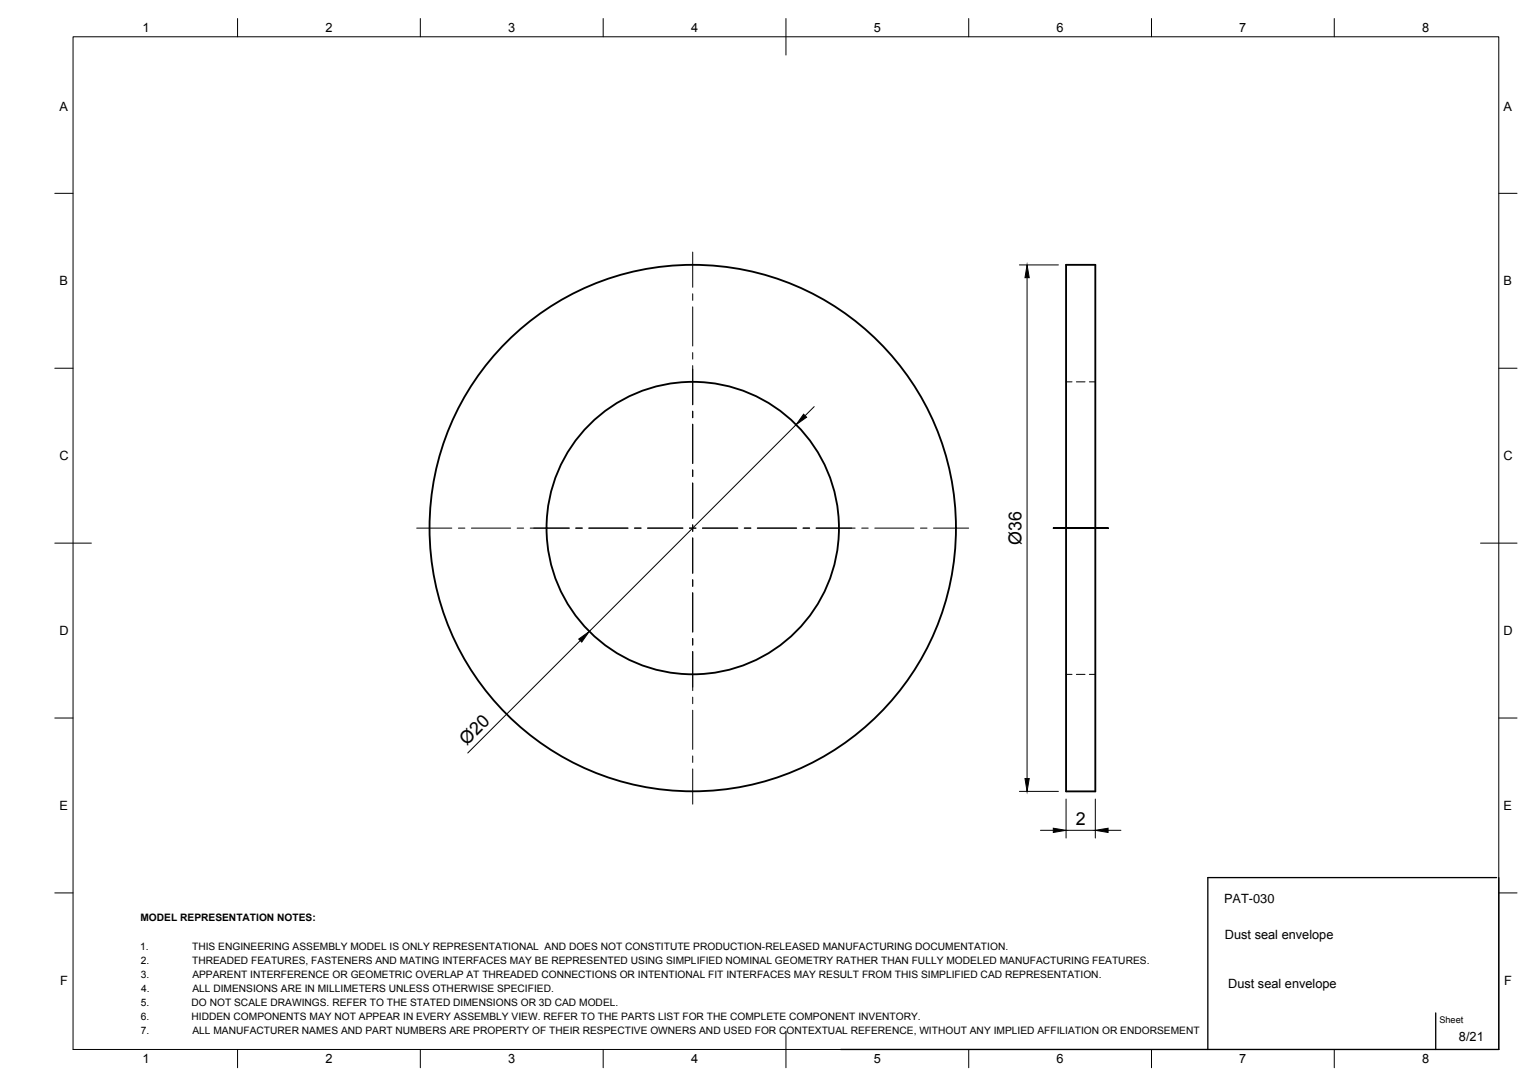
ISO-10303-21;
HEADER;
/* Generated by software containing ST-Developer
 * from STEP Tools, Inc. (www.steptools.com) 
 */

FILE_DESCRIPTION(
/* description */ ('Double-bearing flanged cartridge'),
/* implementation_level */ '2;1');

FILE_NAME(
/* name */ 'Dust seal envelope.step',
/* time_stamp */ '2026-10-28T03:26:40-07:00',
/* author */ (''),
/* organization */ (''),
/* preprocessor_version */ 'ST-DEVELOPER v20.2',
/* originating_system */ 'Autodesk Translation Framework v15.17.0.0',
/* authorisation */ '');

FILE_SCHEMA (('AUTOMOTIVE_DESIGN { 1 0 10303 214 3 1 1 }'));
ENDSEC;

DATA;
#10=MECHANICAL_DESIGN_GEOMETRIC_PRESENTATION_REPRESENTATION('',(#206),#5535);
#170=SHAPE_REPRESENTATION_RELATIONSHIP('SRR','None',#5612,#184);
#184=ADVANCED_BREP_SHAPE_REPRESENTATION('',(#228),#5528);
#206=STYLED_ITEM('',(#5771),#228);
#228=MANIFOLD_SOLID_BREP('Body1',#2340);
#276=FACE_BOUND('',#651,.T.);
#277=FACE_BOUND('',#653,.T.);
#335=PLANE('',#2744);
#336=PLANE('',#2745);
#456=FACE_OUTER_BOUND('',#648,.T.);
#457=FACE_OUTER_BOUND('',#649,.T.);
#458=FACE_OUTER_BOUND('',#650,.T.);
#459=FACE_OUTER_BOUND('',#652,.T.);
#648=EDGE_LOOP('',(#1918,#1919,#1920,#1921));
#649=EDGE_LOOP('',(#1922,#1923,#1924,#1925));
#650=EDGE_LOOP('',(#1926));
#651=EDGE_LOOP('',(#1927));
#652=EDGE_LOOP('',(#1928));
#653=EDGE_LOOP('',(#1929));
#768=LINE('',#4453,#854);
#769=LINE('',#4459,#855);
#854=VECTOR('',#3385,1.);
#855=VECTOR('',#3392,1.8);
#1022=CIRCLE('',#2739,1.);
#1023=CIRCLE('',#2740,1.);
#1024=CIRCLE('',#2742,1.8);
#1025=CIRCLE('',#2743,1.8);
#1204=VERTEX_POINT('',#4450);
#1205=VERTEX_POINT('',#4452);
#1206=VERTEX_POINT('',#4456);
#1207=VERTEX_POINT('',#4458);
#1452=EDGE_CURVE('',#1204,#1204,#1022,.T.);
#1453=EDGE_CURVE('',#1204,#1205,#768,.T.);
#1454=EDGE_CURVE('',#1205,#1205,#1023,.T.);
#1455=EDGE_CURVE('',#1206,#1206,#1024,.T.);
#1456=EDGE_CURVE('',#1206,#1207,#769,.T.);
#1457=EDGE_CURVE('',#1207,#1207,#1025,.T.);
#1918=ORIENTED_EDGE('',*,*,#1452,.F.);
#1919=ORIENTED_EDGE('',*,*,#1453,.T.);
#1920=ORIENTED_EDGE('',*,*,#1454,.T.);
#1921=ORIENTED_EDGE('',*,*,#1453,.F.);
#1922=ORIENTED_EDGE('',*,*,#1455,.F.);
#1923=ORIENTED_EDGE('',*,*,#1456,.T.);
#1924=ORIENTED_EDGE('',*,*,#1457,.T.);
#1925=ORIENTED_EDGE('',*,*,#1456,.F.);
#1926=ORIENTED_EDGE('',*,*,#1455,.T.);
#1927=ORIENTED_EDGE('',*,*,#1452,.T.);
#1928=ORIENTED_EDGE('',*,*,#1457,.F.);
#1929=ORIENTED_EDGE('',*,*,#1454,.F.);
#2152=CYLINDRICAL_SURFACE('',#2738,1.);
#2153=CYLINDRICAL_SURFACE('',#2741,1.8);
#2270=ADVANCED_FACE('',(#456),#2152,.F.);
#2271=ADVANCED_FACE('',(#457),#2153,.T.);
#2272=ADVANCED_FACE('',(#458,#276),#335,.T.);
#2273=ADVANCED_FACE('',(#459,#277),#336,.F.);
#2340=CLOSED_SHELL('',(#2270,#2271,#2272,#2273));
#2737=AXIS2_PLACEMENT_3D('',#4448,#3379,#3380);
#2738=AXIS2_PLACEMENT_3D('',#4449,#3381,#3382);
#2739=AXIS2_PLACEMENT_3D('',#4451,#3383,#3384);
#2740=AXIS2_PLACEMENT_3D('',#4454,#3386,#3387);
#2741=AXIS2_PLACEMENT_3D('',#4455,#3388,#3389);
#2742=AXIS2_PLACEMENT_3D('',#4457,#3390,#3391);
#2743=AXIS2_PLACEMENT_3D('',#4460,#3393,#3394);
#2744=AXIS2_PLACEMENT_3D('',#4461,#3395,#3396);
#2745=AXIS2_PLACEMENT_3D('',#4462,#3397,#3398);
#3379=DIRECTION('axis',(0.,0.,1.));
#3380=DIRECTION('refdir',(1.,0.,0.));
#3381=DIRECTION('center_axis',(0.,1.,0.));
#3382=DIRECTION('ref_axis',(1.,0.,0.));
#3383=DIRECTION('center_axis',(0.,-1.,0.));
#3384=DIRECTION('ref_axis',(1.,0.,0.));
#3385=DIRECTION('',(0.,-1.,0.));
#3386=DIRECTION('center_axis',(0.,-1.,0.));
#3387=DIRECTION('ref_axis',(1.,0.,0.));
#3388=DIRECTION('center_axis',(0.,1.,0.));
#3389=DIRECTION('ref_axis',(1.,0.,0.));
#3390=DIRECTION('center_axis',(0.,1.,0.));
#3391=DIRECTION('ref_axis',(1.,0.,0.));
#3392=DIRECTION('',(0.,-1.,0.));
#3393=DIRECTION('center_axis',(0.,1.,0.));
#3394=DIRECTION('ref_axis',(1.,0.,0.));
#3395=DIRECTION('center_axis',(0.,1.,0.));
#3396=DIRECTION('ref_axis',(1.,0.,0.));
#3397=DIRECTION('center_axis',(0.,1.,0.));
#3398=DIRECTION('ref_axis',(1.,0.,0.));
#4448=CARTESIAN_POINT('',(0.,0.,0.));
#4449=CARTESIAN_POINT('Origin',(0.,-0.4,4.5));
#4450=CARTESIAN_POINT('',(-1.,-0.2,4.5));
#4451=CARTESIAN_POINT('Origin',(0.,-0.2,4.5));
#4452=CARTESIAN_POINT('',(-1.,-0.4,4.5));
#4453=CARTESIAN_POINT('',(-1.,-0.4,4.5));
#4454=CARTESIAN_POINT('Origin',(0.,-0.4,4.5));
#4455=CARTESIAN_POINT('Origin',(0.,-0.4,4.5));
#4456=CARTESIAN_POINT('',(-1.8,-0.2,4.5));
#4457=CARTESIAN_POINT('Origin',(0.,-0.2,4.5));
#4458=CARTESIAN_POINT('',(-1.8,-0.4,4.5));
#4459=CARTESIAN_POINT('',(-1.8,-0.4,4.5));
#4460=CARTESIAN_POINT('Origin',(0.,-0.4,4.5));
#4461=CARTESIAN_POINT('Origin',(0.,-0.2,4.5));
#4462=CARTESIAN_POINT('Origin',(0.,-0.4,4.5));
#5509=UNCERTAINTY_MEASURE_WITH_UNIT(LENGTH_MEASURE(0.001),#5536,
'DISTANCE_ACCURACY_VALUE',
'Maximum model space distance between geometric entities at asserted c
onnectivities');
#5516=UNCERTAINTY_MEASURE_WITH_UNIT(LENGTH_MEASURE(0.001),#5536,
'DISTANCE_ACCURACY_VALUE',
'Maximum model space distance between geometric entities at asserted c
onnectivities');
#5528=(
GEOMETRIC_REPRESENTATION_CONTEXT(3)
GLOBAL_UNCERTAINTY_ASSIGNED_CONTEXT((#5509))
GLOBAL_UNIT_ASSIGNED_CONTEXT((#5536,#5538,#5539))
REPRESENTATION_CONTEXT('','3D')
);
#5535=(
GEOMETRIC_REPRESENTATION_CONTEXT(3)
GLOBAL_UNCERTAINTY_ASSIGNED_CONTEXT((#5516))
GLOBAL_UNIT_ASSIGNED_CONTEXT((#5536,#5538,#5539))
REPRESENTATION_CONTEXT('','3D')
);
#5536=(
LENGTH_UNIT()
NAMED_UNIT(*)
SI_UNIT(.CENTI.,.METRE.)
);
#5538=(
NAMED_UNIT(*)
PLANE_ANGLE_UNIT()
SI_UNIT($,.RADIAN.)
);
#5539=(
NAMED_UNIT(*)
SI_UNIT($,.STERADIAN.)
SOLID_ANGLE_UNIT()
);
#5551=SHAPE_DEFINITION_REPRESENTATION(#5574,#5612);
#5574=PRODUCT_DEFINITION_SHAPE('',$,#5631);
#5612=SHAPE_REPRESENTATION('',(#2737),#5528);
#5619=PRODUCT_DEFINITION_CONTEXT('part definition',#5675,'design');
#5631=PRODUCT_DEFINITION('Dust seal envelope','Dust seal envelope',#5649,
#5619);
#5649=PRODUCT_DEFINITION_FORMATION('',$,#5688);
#5675=APPLICATION_CONTEXT(
'Core Data for Automotive Mechanical Design Process');
#5676=PRODUCT_CONTEXT('part definition',#5675,'mechanical');
#5688=PRODUCT('Dust seal envelope','Dust seal envelope',
'Dust seal envelope',(#5676));
#5765=COLOUR_RGB('Black',0.12,0.14,0.17);
#5766=FILL_AREA_STYLE_COLOUR('',#5765);
#5767=FILL_AREA_STYLE('',(#5766));
#5768=SURFACE_STYLE_FILL_AREA(#5767);
#5769=SURFACE_SIDE_STYLE('',(#5768));
#5770=SURFACE_STYLE_USAGE(.BOTH.,#5769);
#5771=PRESENTATION_STYLE_ASSIGNMENT((#5770));
ENDSEC;
END-ISO-10303-21;
